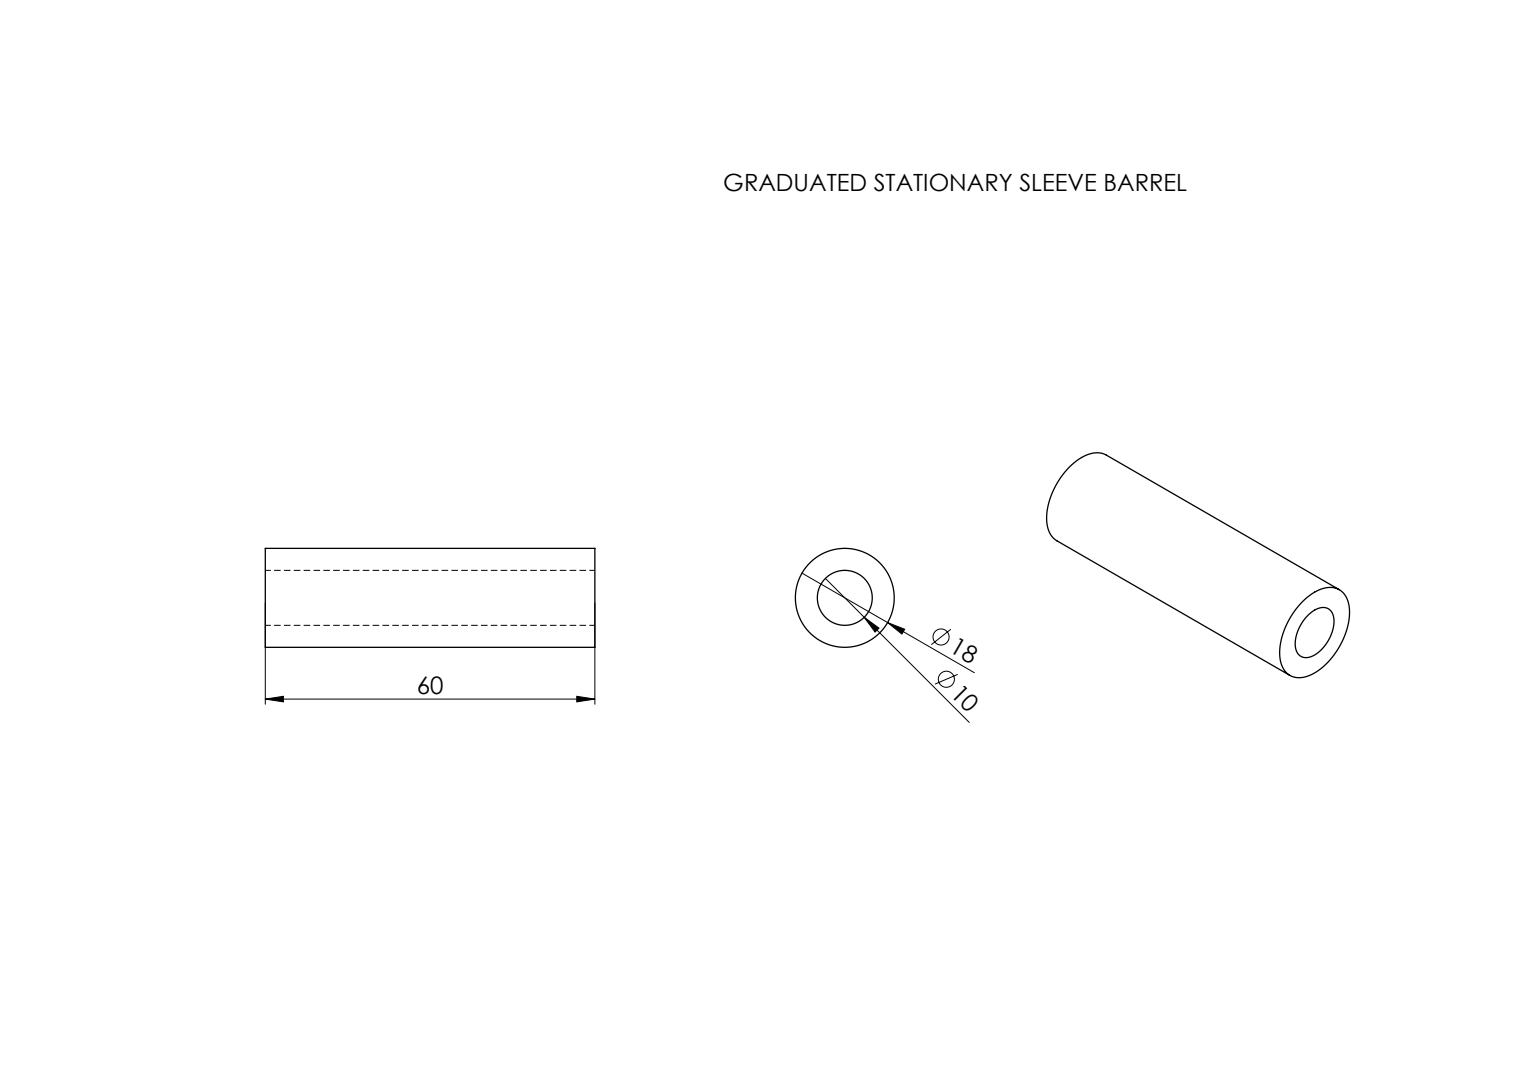
ISO-10303-21;
HEADER;
FILE_DESCRIPTION (('STEP AP214'),
    '1' );
FILE_NAME ('Graduated Stationary Sleeve Barrel.step',
    '2026-10-22T12:35:56',
    ( '' ),
    ( '' ),
    'SwSTEP 2.0',
    'SolidWorks 2026',
    '' );
FILE_SCHEMA (( 'AUTOMOTIVE_DESIGN' ));
ENDSEC;

DATA;
#3=EDGE_CURVE ( 'NONE', #403, #2721, #1745, .T. ) ;
#11=ORIENTED_EDGE ( 'NONE', *, *, #1483, .T. ) ;
#14=VECTOR ( 'NONE', #2502, 1000.000000000000000 ) ;
#17=DIRECTION ( 'NONE',  ( -0.000000000000000000, -0.000000000000000000, 1.000000000000000000 ) ) ;
#30=ORIENTED_EDGE ( 'NONE', *, *, #3, .T. ) ;
#34=DIRECTION ( 'NONE',  ( 1.000000000000000000, 2.312964634635742957E-16, 0.000000000000000000 ) ) ;
#36=CIRCLE ( 'NONE', #2432, 1.500000000000001332 ) ;
#39=DIRECTION ( 'NONE',  ( -0.000000000000000000, -0.000000000000000000, 1.000000000000000000 ) ) ;
#46=DIRECTION ( 'NONE',  ( 1.000000000000000000, 0.000000000000000000, 0.000000000000000000 ) ) ;
#48=DIRECTION ( 'NONE',  ( 0.000000000000000000, 1.000000000000000000, 0.000000000000000000 ) ) ;
#53=AXIS2_PLACEMENT_3D ( 'NONE', #2212, #1162, #2179 ) ;
#55=DIRECTION ( 'NONE',  ( -0.000000000000000000, -0.000000000000000000, 1.000000000000000000 ) ) ;
#113=DIRECTION ( 'NONE',  ( 1.000000000000000000, 0.000000000000000000, 0.000000000000000000 ) ) ;
#126=CARTESIAN_POINT ( 'NONE',  ( 38.49999999999999289, 1.474514954580286030E-14, 20.99999999999999645 ) ) ;
#133=APPLICATION_CONTEXT ( 'automotive_design' ) ;
#140=CONICAL_SURFACE ( 'NONE', #2380, 1.250000000000001110, 1.029744258676654090 ) ;
#143=CARTESIAN_POINT ( 'NONE',  ( 38.49999999999997868, 0.1985404316418196702, 16.49999999999998224 ) ) ;
#159=ORIENTED_EDGE ( 'NONE', *, *, #497, .T. ) ;
#161=AXIS2_PLACEMENT_3D ( 'NONE', #1164, #1184, #2943 ) ;
#164=FACE_OUTER_BOUND ( 'NONE', #1049, .T. ) ;
#165=ADVANCED_FACE ( 'NONE', ( #2345 ), #2393, .F. ) ;
#185=DIRECTION ( 'NONE',  ( -0.000000000000000000, -0.000000000000000000, 1.000000000000000000 ) ) ;
#191=( NAMED_UNIT ( * ) PLANE_ANGLE_UNIT ( ) SI_UNIT ( $, .RADIAN. ) );
#196=CARTESIAN_POINT ( 'NONE',  ( 35.50000000000000000, 0.1959257125632855590, 16.50000000000000000 ) ) ;
#197=ORIENTED_EDGE ( 'NONE', *, *, #540, .T. ) ;
#235=CARTESIAN_POINT ( 'NONE',  ( 38.45202114561162432, -0.3888602178275583632, 16.49210820886665374 ) ) ;
#237=CARTESIAN_POINT ( 'NONE',  ( 37.21237719682158485, -0.3527350612243344563, 12.48805154969246978 ) ) ;
#241=VERTEX_POINT ( 'NONE', #734 ) ;
#262=ORIENTED_EDGE ( 'NONE', *, *, #615, .T. ) ;
#264=EDGE_LOOP ( 'NONE', ( #371, #711 ) ) ;
#267=CARTESIAN_POINT ( 'NONE',  ( 36.63069504892280293, -0.2100771151993728880, 12.49609970571322570 ) ) ;
#268=AXIS2_PLACEMENT_3D ( 'NONE', #899, #2909, #681 ) ;
#269=CYLINDRICAL_SURFACE ( 'NONE', #1531, 1.250000000000001110 ) ;
#275=LINE ( 'NONE', #3009, #3087 ) ;
#293=ORIENTED_EDGE ( 'NONE', *, *, #2633, .T. ) ;
#294=DIRECTION ( 'NONE',  ( 1.000000000000000000, 0.000000000000000000, 0.000000000000000000 ) ) ;
#301=AXIS2_PLACEMENT_3D ( 'NONE', #323, #2823, #614 ) ;
#302=FACE_OUTER_BOUND ( 'NONE', #2160, .T. ) ;
#310=VERTEX_POINT ( 'NONE', #723 ) ;
#312=CARTESIAN_POINT ( 'NONE',  ( 37.00000000000000000, 1.474514954580286030E-14, 20.99999999999999645 ) ) ;
#318=DIRECTION ( 'NONE',  ( -1.000000000000000000, -0.000000000000000000, -0.000000000000000000 ) ) ;
#323=CARTESIAN_POINT ( 'NONE',  ( 87.00000000000000000, -7.622732162557277534E-15, 7.500000000000000000 ) ) ;
#326=VECTOR ( 'NONE', #1980, 1000.000000000000000 ) ;
#331=CARTESIAN_POINT ( 'NONE',  ( 27.00000000000000000, -7.622732162557277534E-15, 7.500000000000000000 ) ) ;
#365=CARTESIAN_POINT ( 'NONE',  ( 35.65194399346783882, -0.6651260505907211629, 16.47584948644689007 ) ) ;
#371=ORIENTED_EDGE ( 'NONE', *, *, #1189, .F. ) ;
#375=DIRECTION ( 'NONE',  ( -0.000000000000000000, -0.000000000000000000, 1.000000000000000000 ) ) ;
#379=ORIENTED_EDGE ( 'NONE', *, *, #1424, .F. ) ;
#403=VERTEX_POINT ( 'NONE', #1979 ) ;
#408=DIRECTION ( 'NONE',  ( 1.000000000000000000, 0.000000000000000000, 0.000000000000000000 ) ) ;
#416=CARTESIAN_POINT ( 'NONE',  ( 35.50000000000000000, -7.622732095468789599E-15, 16.49999999999999289 ) ) ;
#419=UNCERTAINTY_MEASURE_WITH_UNIT (LENGTH_MEASURE( 1.000000000000000082E-05 ), #2203, 'distance_accuracy_value', 'NONE');
#422=CARTESIAN_POINT ( 'NONE',  ( 38.49999999999999289, -7.622732162557277534E-15, 16.49999999999999289 ) ) ;
#423=DIRECTION ( 'NONE',  ( -3.854941057726241055E-16, 1.000000000000000000, 0.000000000000000000 ) ) ;
#429=CARTESIAN_POINT ( 'NONE',  ( 37.09819064725438409, 1.500059831078516703, 16.37410956135321882 ) ) ;
#432=ORIENTED_EDGE ( 'NONE', *, *, #882, .F. ) ;
#448=CARTESIAN_POINT ( 'NONE',  ( 38.19805860116023410, 0.9234461779904211687, 16.45357685834586903 ) ) ;
#458=( NAMED_UNIT ( * ) SI_UNIT ( $, .STERADIAN. ) SOLID_ANGLE_UNIT ( ) );
#463=DIRECTION ( 'NONE',  ( -0.000000000000000000, -0.000000000000000000, 1.000000000000000000 ) ) ;
#468=CARTESIAN_POINT ( 'NONE',  ( 38.12949724085409287, -0.9918543271721246279, 16.44544909559323287 ) ) ;
#475=ADVANCED_FACE ( 'NONE', ( #1758, #2466 ), #1952, .F. ) ;
#478=EDGE_LOOP ( 'NONE', ( #2640, #2192 ) ) ;
#481=B_SPLINE_CURVE_WITH_KNOTS ( 'NONE', 3,
 ( #609, #3129, #1643, #1588, #2584, #1338, #1883, #2554, #896, #1864 ),
 .UNSPECIFIED., .F., .F.,
 ( 4, 2, 2, 2, 4 ),
 ( 0.0002158803543021033892, 0.0005338002860526318500, 0.0008517202178031603108, 0.001169640149553688880, 0.001487560081304217232 ),
 .UNSPECIFIED. ) ;
#484=DIRECTION ( 'NONE',  ( 1.000000000000000000, 0.000000000000000000, 0.000000000000000000 ) ) ;
#489=STYLED_ITEM('',(#3271),#1054);
#497=EDGE_CURVE ( 'NONE', #2088, #3100, #2946, .T. ) ;
#507=EDGE_LOOP ( 'NONE', ( #1692, #1273, #197, #3052 ) ) ;
#512=CIRCLE ( 'NONE', #301, 8.999999999999992895 ) ;
#518=CARTESIAN_POINT ( 'NONE',  ( 38.34772064623945198, -0.6658172387807467230, 16.47579882838004295 ) ) ;
#531=VERTEX_POINT ( 'NONE', #845 ) ;
#535=VECTOR ( 'NONE', #185, 1000.000000000000000 ) ;
#540=EDGE_CURVE ( 'NONE', #2776, #241, #816, .T. ) ;
#551=AXIS2_PLACEMENT_3D ( 'NONE', #3000, #773, #2215 ) ;
#552=CARTESIAN_POINT ( 'NONE',  ( 35.80758137781342043, -0.9152444266664223615, 16.45371270176149991 ) ) ;
#567=DIRECTION ( 'NONE',  ( 0.000000000000000000, 0.000000000000000000, 1.000000000000000000 ) ) ;
#573=LINE ( 'NONE', #2313, #957 ) ;
#589=ORIENTED_EDGE ( 'NONE', *, *, #610, .T. ) ;
#603=( GEOMETRIC_REPRESENTATION_CONTEXT ( 3 ) GLOBAL_UNCERTAINTY_ASSIGNED_CONTEXT ( ( #419 ) ) GLOBAL_UNIT_ASSIGNED_CONTEXT ( ( #2203, #1706, #998 ) ) REPRESENTATION_CONTEXT ( 'NONE', 'WORKASPACE' ) );
#607=ORIENTED_EDGE ( 'NONE', *, *, #667, .F. ) ;
#609=CARTESIAN_POINT ( 'NONE',  ( 36.58213974117523293, -6.323013916343274967E-15, 12.50000000000000178 ) ) ;
#610=EDGE_CURVE ( 'NONE', #531, #1119, #1170, .T. ) ;
#611=ORIENTED_EDGE ( 'NONE', *, *, #718, .T. ) ;
#614=DIRECTION ( 'NONE',  ( 0.000000000000000000, 1.000000000000000000, 0.000000000000000000 ) ) ;
#615=EDGE_CURVE ( 'NONE', #1621, #241, #2725, .T. ) ;
#618=CIRCLE ( 'NONE', #2483, 5.000000000000000000 ) ;
#621=CARTESIAN_POINT ( 'NONE',  ( 36.58213974117523293, -6.323013916343274967E-15, 12.50000000000000178 ) ) ;
#625=CARTESIAN_POINT ( 'NONE',  ( 37.38775466693719807, 1.452318184980633031, 16.38206869443958169 ) ) ;
#630=VECTOR ( 'NONE', #2703, 1000.000000000000000 ) ;
#637=ADVANCED_FACE ( 'NONE', ( #2299 ), #812, .F. ) ;
#655=CARTESIAN_POINT ( 'NONE',  ( 37.00000000000000000, 1.474514954580286030E-14, 12.99999999999999822 ) ) ;
#661=ORIENTED_EDGE ( 'NONE', *, *, #1385, .F. ) ;
#667=EDGE_CURVE ( 'NONE', #531, #3100, #2993, .T. ) ;
#669=ORIENTED_EDGE ( 'NONE', *, *, #1688, .T. ) ;
#674=CARTESIAN_POINT ( 'NONE',  ( 87.00000000000000000, -7.622732162557277534E-15, 7.500000000000000000 ) ) ;
#676=CARTESIAN_POINT ( 'NONE',  ( 35.68903409116789049, 0.7546922429561601087, 16.47012649564898368 ) ) ;
#677=EDGE_CURVE ( 'NONE', #861, #1621, #573, .T. ) ;
#681=DIRECTION ( 'NONE',  ( 0.000000000000000000, 1.000000000000000000, 0.000000000000000000 ) ) ;
#689=CARTESIAN_POINT ( 'NONE',  ( 35.50000000000000000, -7.622732095468789599E-15, 16.49999999999999289 ) ) ;
#691=ORIENTED_EDGE ( 'NONE', *, *, #1656, .T. ) ;
#696=CARTESIAN_POINT ( 'NONE',  ( 87.00000000000000000, -7.010408762983600216E-15, 2.499999999999999556 ) ) ;
#699=CLOSED_SHELL ( 'NONE', ( #2287, #1331, #2040, #2558, #1386, #1530, #475, #2835, #165, #637, #795, #1234, #1613 ) ) ;
#704=VECTOR ( 'NONE', #1350, 1000.000000000000000 ) ;
#709=ORIENTED_EDGE ( 'NONE', *, *, #2679, .T. ) ;
#711=ORIENTED_EDGE ( 'NONE', *, *, #1812, .F. ) ;
#718=EDGE_CURVE ( 'NONE', #310, #1076, #275, .T. ) ;
#722=AXIS2_PLACEMENT_3D ( 'NONE', #2605, #1834, #113 ) ;
#723=CARTESIAN_POINT ( 'NONE',  ( 87.00000000000000000, -6.520550043324660412E-15, -1.499999999999992673 ) ) ;
#734=CARTESIAN_POINT ( 'NONE',  ( 38.25000000000000000, 1.474514954580286030E-14, 12.99999999999999822 ) ) ;
#739=AXIS2_PLACEMENT_3D ( 'NONE', #3054, #318, #567 ) ;
#742=CARTESIAN_POINT ( 'NONE',  ( 37.36887240208277916, -0.2104090322588208772, 12.49607929530250239 ) ) ;
#751=AXIS2_PLACEMENT_3D ( 'NONE', #312, #39, #294 ) ;
#757=PLANE ( 'NONE',  #2282 ) ;
#764=DIRECTION ( 'NONE',  ( 1.000000000000000000, 0.000000000000000000, 0.000000000000000000 ) ) ;
#766=DIRECTION ( 'NONE',  ( 1.000000000000000000, 0.000000000000000000, 0.000000000000000000 ) ) ;
#768=ORIENTED_EDGE ( 'NONE', *, *, #610, .F. ) ;
#773=DIRECTION ( 'NONE',  ( 1.000000000000000000, 2.312964634635742957E-16, 0.000000000000000000 ) ) ;
#775=DIRECTION ( 'NONE',  ( 1.000000000000000000, 0.000000000000000000, 0.000000000000000000 ) ) ;
#787=CARTESIAN_POINT ( 'NONE',  ( 37.41786025882473865, -0.1064896851603509553, 12.50000000000000178 ) ) ;
#795=ADVANCED_FACE ( 'NONE', ( #2578 ), #1099, .F. ) ;
#797=CIRCLE ( 'NONE', #2874, 8.999999999999992895 ) ;
#805=CARTESIAN_POINT ( 'NONE',  ( 35.75000000000000000, 1.489823039569627924E-14, 13.99999999999999822 ) ) ;
#809=COLOUR_RGB ( '',0.8941176470588234615, 0.8941176470588234615, 0.8941176470588234615 ) ;
#812=CYLINDRICAL_SURFACE ( 'NONE', #751, 1.499999999999994449 ) ;
#816=LINE ( 'NONE', #3033, #704 ) ;
#817=AXIS2_PLACEMENT_3D ( 'NONE', #2148, #3132, #1968 ) ;
#819=ORIENTED_EDGE ( 'NONE', *, *, #1576, .T. ) ;
#832=LINE ( 'NONE', #2833, #2937 ) ;
#838=LINE ( 'NONE', #2784, #2614 ) ;
#845=CARTESIAN_POINT ( 'NONE',  ( 35.50000000000000000, 1.492884656567496302E-14, 13.99999999999999822 ) ) ;
#847=ORIENTED_EDGE ( 'NONE', *, *, #1892, .F. ) ;
#850=AXIS2_PLACEMENT_3D ( 'NONE', #2539, #2547, #764 ) ;
#851=FACE_OUTER_BOUND ( 'NONE', #1488, .T. ) ;
#854=EDGE_LOOP ( 'NONE', ( #691, #589 ) ) ;
#858=EDGE_LOOP ( 'NONE', ( #30, #819 ) ) ;
#861=VERTEX_POINT ( 'NONE', #621 ) ;
#868=ORIENTED_EDGE ( 'NONE', *, *, #2571, .F. ) ;
#870=ORIENTED_EDGE ( 'NONE', *, *, #1061, .T. ) ;
#875=EDGE_LOOP ( 'NONE', ( #768, #1279, #2791, #1807 ) ) ;
#876=CARTESIAN_POINT ( 'NONE',  ( 38.49999999999999289, -7.622732162557277534E-15, 16.49999999999999289 ) ) ;
#882=EDGE_CURVE ( 'NONE', #1076, #1030, #797, .T. ) ;
#896=CARTESIAN_POINT ( 'NONE',  ( 37.41786025882475286, 0.1065494216233999342, 12.50000000000000000 ) ) ;
#898=CIRCLE ( 'NONE', #1363, 5.000000000000000000 ) ;
#899=CARTESIAN_POINT ( 'NONE',  ( 87.00000000000000000, -7.622732162557277534E-15, 7.500000000000000000 ) ) ;
#902=CARTESIAN_POINT ( 'NONE',  ( 87.00000000000000000, -7.622732162557277534E-15, 12.50000000000000000 ) ) ;
#906=AXIS2_PLACEMENT_3D ( 'NONE', #1555, #2527, #46 ) ;
#913=LINE ( 'NONE', #126, #3161 ) ;
#919=DIRECTION ( 'NONE',  ( -1.000000000000000000, -0.000000000000000000, -0.000000000000000000 ) ) ;
#932=ORIENTED_EDGE ( 'NONE', *, *, #1576, .F. ) ;
#939=AXIS2_PLACEMENT_3D ( 'NONE', #1517, #463, #766 ) ;
#942=CARTESIAN_POINT ( 'NONE',  ( 38.45998082922277916, 0.3957415549423320411, 16.49311123862705486 ) ) ;
#949=CARTESIAN_POINT ( 'NONE',  ( 38.50000000000000711, -0.09929498707317854778, 16.49999999999999645 ) ) ;
#957=VECTOR ( 'NONE', #1500, 1000.000000000000000 ) ;
#961=ORIENTED_EDGE ( 'NONE', *, *, #2571, .T. ) ;
#976=CARTESIAN_POINT ( 'NONE',  ( 38.30162487582175856, -0.7519129166725451174, 16.46890859085320002 ) ) ;
#982=( LENGTH_UNIT ( ) NAMED_UNIT ( * ) SI_UNIT ( .MILLI., .METRE. ) );
#993=FACE_OUTER_BOUND ( 'NONE', #854, .T. ) ;
#998=( NAMED_UNIT ( * ) SI_UNIT ( $, .STERADIAN. ) SOLID_ANGLE_UNIT ( ) );
#999=ORIENTED_EDGE ( 'NONE', *, *, #2679, .F. ) ;
#1011=EDGE_LOOP ( 'NONE', ( #607, #1544, #1039, #1313 ) ) ;
#1015=CARTESIAN_POINT ( 'NONE',  ( 37.41786025882474576, -7.616137346557303354E-15, 12.50000000000000000 ) ) ;
#1027=CARTESIAN_POINT ( 'NONE',  ( 35.69898883018242230, -0.7529305858385405559, 16.46882038169669471 ) ) ;
#1030=VERTEX_POINT ( 'NONE', #1461 ) ;
#1032=CARTESIAN_POINT ( 'NONE',  ( 38.50000000000000000, 1.474514954580286030E-14, 13.99999999999999822 ) ) ;
#1037=FACE_OUTER_BOUND ( 'NONE', #875, .T. ) ;
#1039=ORIENTED_EDGE ( 'NONE', *, *, #1721, .T. ) ;
#1049=EDGE_LOOP ( 'NONE', ( #11, #3163, #2385, #847, #2923, #379 ) ) ;
#1054=MANIFOLD_SOLID_BREP ( 'Boss-Extrude1', #699 ) ;
#1061=EDGE_CURVE ( 'NONE', #1916, #1595, #898, .T. ) ;
#1062=CARTESIAN_POINT ( 'NONE',  ( 36.24410157368014751, -1.310477515365985557, 16.40440676504733730 ) ) ;
#1073=CARTESIAN_POINT ( 'NONE',  ( 36.80294994545205611, -1.490236770648107001, 16.37578575999040353 ) ) ;
#1076=VERTEX_POINT ( 'NONE', #2035 ) ;
#1094=CIRCLE ( 'NONE', #161, 8.999999999999992895 ) ;
#1099=CONICAL_SURFACE ( 'NONE', #2559, 1.250000000000001110, 1.029744258676654090 ) ;
#1114=CYLINDRICAL_SURFACE ( 'NONE', #1861, 1.250000000000001110 ) ;
#1119=VERTEX_POINT ( 'NONE', #1032 ) ;
#1143=ORIENTED_EDGE ( 'NONE', *, *, #1149, .T. ) ;
#1149=EDGE_CURVE ( 'NONE', #310, #2118, #512, .T. ) ;
#1156=ORIENTED_EDGE ( 'NONE', *, *, #2976, .T. ) ;
#1162=DIRECTION ( 'NONE',  ( -1.000000000000000000, -0.000000000000000000, -0.000000000000000000 ) ) ;
#1164=CARTESIAN_POINT ( 'NONE',  ( 27.00000000000000000, -7.622732162557277534E-15, 7.500000000000000000 ) ) ;
#1170=CIRCLE ( 'NONE', #906, 1.500000000000001332 ) ;
#1177=DIRECTION ( 'NONE',  ( 0.000000000000000000, 0.000000000000000000, 1.000000000000000000 ) ) ;
#1179=CARTESIAN_POINT ( 'NONE',  ( 35.80050950286611311, 0.9216565616594220023, 16.45376772233409923 ) ) ;
#1184=DIRECTION ( 'NONE',  ( 1.000000000000000000, 2.312964634635742957E-16, 0.000000000000000000 ) ) ;
#1188=CIRCLE ( 'NONE', #2903, 5.000000000000000000 ) ;
#1189=EDGE_CURVE ( 'NONE', #2624, #2847, #1600, .T. ) ;
#1193=CARTESIAN_POINT ( 'NONE',  ( 36.60604563826974811, 1.460666791800832254, 16.38100777177577072 ) ) ;
#1217=FILL_AREA_STYLE ('',( #1245 ) ) ;
#1228=CARTESIAN_POINT ( 'NONE',  ( 37.39427925860091051, -1.460378464396907328, 16.38104908776753632 ) ) ;
#1230=CARTESIAN_POINT ( 'NONE',  ( 37.10670076043889765, -0.3922264638554286975, 12.48459209977295181 ) ) ;
#1234=ADVANCED_FACE ( 'NONE', ( #851 ), #1114, .F. ) ;
#1244=( NAMED_UNIT ( * ) PLANE_ANGLE_UNIT ( ) SI_UNIT ( $, .RADIAN. ) );
#1245=FILL_AREA_STYLE_COLOUR ( '', #809 ) ;
#1257=CARTESIAN_POINT ( 'NONE',  ( 37.00000000000000000, 1.474514954580286030E-14, 20.99999999999999645 ) ) ;
#1266=DIRECTION ( 'NONE',  ( -1.000000000000000000, -0.000000000000000000, -0.000000000000000000 ) ) ;
#1273=ORIENTED_EDGE ( 'NONE', *, *, #2997, .T. ) ;
#1279=ORIENTED_EDGE ( 'NONE', *, *, #667, .T. ) ;
#1288=CIRCLE ( 'NONE', #2072, 1.250000000000001110 ) ;
#1313=ORIENTED_EDGE ( 'NONE', *, *, #1688, .F. ) ;
#1322=CARTESIAN_POINT ( 'NONE',  ( 35.57671993710910385, -0.4836543419624433349, 16.48745487577124180 ) ) ;
#1331=ADVANCED_FACE ( 'NONE', ( #2709 ), #140, .F. ) ;
#1336=CARTESIAN_POINT ( 'NONE',  ( 36.90254329834229452, -1.500037116461185871, 16.37411340082286770 ) ) ;
#1338=CARTESIAN_POINT ( 'NONE',  ( 37.10600482971271674, 0.3921370382570182889, 12.48459913632445506 ) ) ;
#1347=DIRECTION ( 'NONE',  ( -1.000000000000000000, -0.000000000000000000, -0.000000000000000000 ) ) ;
#1350=DIRECTION ( 'NONE',  ( 0.8571673007021121116, 0.000000000000000000, 0.5150380749100544886 ) ) ;
#1363=AXIS2_PLACEMENT_3D ( 'NONE', #2734, #2249, #1546 ) ;
#1385=EDGE_CURVE ( 'NONE', #1916, #2721, #1937, .T. ) ;
#1386=ADVANCED_FACE ( 'NONE', ( #2199 ), #1426, .T. ) ;
#1390=CARTESIAN_POINT ( 'NONE',  ( 35.75000000000000000, 1.489823039569627924E-14, 20.99999999999999645 ) ) ;
#1399=CARTESIAN_POINT ( 'NONE',  ( 36.24736826332971162, 1.301195037071590122, 16.40561087244777028 ) ) ;
#1416=CARTESIAN_POINT ( 'NONE',  ( 35.53942839536622955, 0.3936020622859700002, 16.49320894598176679 ) ) ;
#1420=( GEOMETRIC_REPRESENTATION_CONTEXT ( 3 ) GLOBAL_UNCERTAINTY_ASSIGNED_CONTEXT ( ( #3107 ) ) GLOBAL_UNIT_ASSIGNED_CONTEXT ( ( #982, #1244, #2001 ) ) REPRESENTATION_CONTEXT ( 'NONE', 'WORKASPACE' ) );
#1422=PRODUCT_DEFINITION_CONTEXT ( 'detailed design', #133, 'design' ) ;
#1424=EDGE_CURVE ( 'NONE', #1595, #2776, #3151, .T. ) ;
#1425=LINE ( 'NONE', #1681, #326 ) ;
#1426=CYLINDRICAL_SURFACE ( 'NONE', #817, 8.999999999999994671 ) ;
#1429=CARTESIAN_POINT ( 'NONE',  ( 87.00000000000000000, -7.622732162557277534E-15, 16.49999999999999289 ) ) ;
#1437=ORIENTED_EDGE ( 'NONE', *, *, #2633, .F. ) ;
#1444=SHAPE_REPRESENTATION_RELATIONSHIP ( 'NONE' , 'NONE' ,  #1790, #2267 ) ;
#1461=CARTESIAN_POINT ( 'NONE',  ( 27.00000000000000000, -7.622732162557275957E-15, 16.49999999999999289 ) ) ;
#1470=CARTESIAN_POINT ( 'NONE',  ( 37.75516277711825808, -1.310683246666488833, 16.40437238582925872 ) ) ;
#1479=( LENGTH_UNIT ( ) NAMED_UNIT ( * ) SI_UNIT ( .MILLI., .METRE. ) );
#1483=EDGE_CURVE ( 'NONE', #1595, #1916, #1188, .T. ) ;
#1488=EDGE_LOOP ( 'NONE', ( #868, #2266, #709, #2653 ) ) ;
#1493=CARTESIAN_POINT ( 'NONE',  ( 36.78831377322251228, -0.3533019008417399021, 12.48801788595628892 ) ) ;
#1500=DIRECTION ( 'NONE',  ( -0.8571673007021121116, 1.049727191138618449E-16, 0.5150380749100544886 ) ) ;
#1507=CARTESIAN_POINT ( 'NONE',  ( 38.25000000000000000, 1.474514954580286030E-14, 13.99999999999999822 ) ) ;
#1510=EDGE_CURVE ( 'NONE', #241, #1621, #1288, .T. ) ;
#1517=CARTESIAN_POINT ( 'NONE',  ( 37.00000000000000000, 1.474514954580286030E-14, 13.99999999999999822 ) ) ;
#1518=DIRECTION ( 'NONE',  ( 0.000000000000000000, 1.000000000000000000, 0.000000000000000000 ) ) ;
#1523=FACE_BOUND ( 'NONE', #264, .T. ) ;
#1530=ADVANCED_FACE ( 'NONE', ( #2728, #2969 ), #2530, .T. ) ;
#1531=AXIS2_PLACEMENT_3D ( 'NONE', #1257, #1984, #2971 ) ;
#1544=ORIENTED_EDGE ( 'NONE', *, *, #1656, .F. ) ;
#1546=DIRECTION ( 'NONE',  ( 0.000000000000000000, 1.000000000000000000, 0.000000000000000000 ) ) ;
#1555=CARTESIAN_POINT ( 'NONE',  ( 37.00000000000000000, 1.474514954580286030E-14, 13.99999999999999822 ) ) ;
#1557=DIRECTION ( 'NONE',  ( -0.000000000000000000, -0.000000000000000000, 1.000000000000000000 ) ) ;
#1573=DIRECTION ( 'NONE',  ( -0.000000000000000000, -0.000000000000000000, 1.000000000000000000 ) ) ;
#1576=EDGE_CURVE ( 'NONE', #2721, #403, #618, .T. ) ;
#1577=APPLICATION_CONTEXT ( 'automotive_design' ) ;
#1587=CARTESIAN_POINT ( 'NONE',  ( 36.51683924005256188, -1.423460261948026995, 16.38679996801885252 ) ) ;
#1588=CARTESIAN_POINT ( 'NONE',  ( 36.78802102464440082, 0.3529434585571357696, 12.48803557435225287 ) ) ;
#1595=VERTEX_POINT ( 'NONE', #2790 ) ;
#1600=CIRCLE ( 'NONE', #722, 1.250000000000001110 ) ;
#1601=CARTESIAN_POINT ( 'NONE',  ( 35.49999999999999289, -0.09798730130380635395, 16.49999999999999645 ) ) ;
#1606=EDGE_CURVE ( 'NONE', #2776, #861, #3168, .T. ) ;
#1613=ADVANCED_FACE ( 'NONE', ( #1523, #993 ), #757, .F. ) ;
#1620=CARTESIAN_POINT ( 'NONE',  ( 37.91396272957889124, 1.193436492094938517, 16.42069107455876065 ) ) ;
#1621=VERTEX_POINT ( 'NONE', #3003 ) ;
#1625=DIRECTION ( 'NONE',  ( 1.000000000000000000, 0.000000000000000000, 0.000000000000000000 ) ) ;
#1643=CARTESIAN_POINT ( 'NONE',  ( 36.63137859968045262, 0.2107904407421468673, 12.49606198580778660 ) ) ;
#1647=PRODUCT ( 'Graduated Stationary Sleeve Barrel', 'Graduated Stationary Sleeve Barrel', '', ( #1938 ) ) ;
#1656=EDGE_CURVE ( 'NONE', #1119, #531, #36, .T. ) ;
#1668=DIRECTION ( 'NONE',  ( -1.000000000000000000, -0.000000000000000000, -0.000000000000000000 ) ) ;
#1681=CARTESIAN_POINT ( 'NONE',  ( 38.25000000000000000, 1.474514954580286030E-14, 20.99999999999999645 ) ) ;
#1682=CARTESIAN_POINT ( 'NONE',  ( 87.00000000000000000, -7.622732162557277534E-15, 7.500000000000000000 ) ) ;
#1688=EDGE_CURVE ( 'NONE', #3100, #2088, #1848, .T. ) ;
#1690=CARTESIAN_POINT ( 'NONE',  ( 37.48326775981566072, 1.423407605072616100, 16.38680797912481424 ) ) ;
#1692=ORIENTED_EDGE ( 'NONE', *, *, #677, .F. ) ;
#1706=( NAMED_UNIT ( * ) PLANE_ANGLE_UNIT ( ) SI_UNIT ( $, .RADIAN. ) );
#1721=EDGE_CURVE ( 'NONE', #1119, #2088, #913, .T. ) ;
#1728=CARTESIAN_POINT ( 'NONE',  ( 27.00000000000000000, -7.010408762983600216E-15, 2.499999999999999556 ) ) ;
#1732=ORIENTED_EDGE ( 'NONE', *, *, #1812, .T. ) ;
#1745=CIRCLE ( 'NONE', #1840, 5.000000000000000000 ) ;
#1758=FACE_OUTER_BOUND ( 'NONE', #1816, .T. ) ;
#1760=DIRECTION ( 'NONE',  ( -1.000000000000000000, 0.000000000000000000, -0.000000000000000000 ) ) ;
#1783=DIRECTION ( 'NONE',  ( 1.000000000000000000, 2.312964634635742957E-16, 0.000000000000000000 ) ) ;
#1788=DIRECTION ( 'NONE',  ( 0.000000000000000000, 0.000000000000000000, -1.000000000000000000 ) ) ;
#1790=SHAPE_REPRESENTATION ( 'Graduated Stationary Sleeve Barrel', ( #2878 ), #603 ) ;
#1807=ORIENTED_EDGE ( 'NONE', *, *, #1721, .F. ) ;
#1812=EDGE_CURVE ( 'NONE', #2847, #2624, #2495, .T. ) ;
#1816=EDGE_LOOP ( 'NONE', ( #3075, #432 ) ) ;
#1817=CARTESIAN_POINT ( 'NONE',  ( 36.07902659818449109, -1.200345445641969988, 16.42070378373878725 ) ) ;
#1834=DIRECTION ( 'NONE',  ( -0.000000000000000000, -0.000000000000000000, 1.000000000000000000 ) ) ;
#1837=DIRECTION ( 'NONE',  ( 1.000000000000000000, 0.000000000000000000, 0.000000000000000000 ) ) ;
#1840=AXIS2_PLACEMENT_3D ( 'NONE', #331, #1783, #1518 ) ;
#1848=B_SPLINE_CURVE_WITH_KNOTS ( 'NONE', 3,
 ( #689, #196, #1416, #676, #1179, #1942, #2920, #1399, #2365, #1193, #2652, #429, #2865, #625, #1690, #1930, #2125, #1620, #2190, #448, #3175, #942, #143, #876 ),
 .UNSPECIFIED., .F., .F.,
 ( 4, 2, 2, 2, 2, 2, 2, 2, 2, 2, 2, 4 ),
 ( 0.004697885398315436792, 0.005284974574641427766, 0.005872063750967418741, 0.006165608339130407289, 0.006459152927293394103, 0.007046242103619369465, 0.007339786691782357146, 0.007633331279945343960, 0.007926875868108331641, 0.008220420456271318455, 0.008807509632597295551, 0.009394598808923269179 ),
 .UNSPECIFIED. ) ;
#1861=AXIS2_PLACEMENT_3D ( 'NONE', #1887, #1573, #1625 ) ;
#1864=CARTESIAN_POINT ( 'NONE',  ( 37.41786025882474576, -7.616137346557303354E-15, 12.50000000000000000 ) ) ;
#1873=CYLINDRICAL_SURFACE ( 'NONE', #2446, 1.499999999999994449 ) ;
#1883=CARTESIAN_POINT ( 'NONE',  ( 37.21226234515645359, 0.3528290111407958451, 12.48804596179740756 ) ) ;
#1887=CARTESIAN_POINT ( 'NONE',  ( 37.00000000000000000, 1.474514954580286030E-14, 20.99999999999999645 ) ) ;
#1892=EDGE_CURVE ( 'NONE', #861, #403, #2205, .T. ) ;
#1897=ORIENTED_EDGE ( 'NONE', *, *, #540, .F. ) ;
#1914=ORIENTED_EDGE ( 'NONE', *, *, #718, .F. ) ;
#1916=VERTEX_POINT ( 'NONE', #2962 ) ;
#1920=UNCERTAINTY_MEASURE_WITH_UNIT (LENGTH_MEASURE( 1.000000000000000082E-05 ), #1479, 'distance_accuracy_value', 'NONE');
#1930=CARTESIAN_POINT ( 'NONE',  ( 37.66466167501430107, 1.348281052163445404, 16.39851580165995415 ) ) ;
#1932=EDGE_LOOP ( 'NONE', ( #2500, #2163, #262, #1897 ) ) ;
#1937=LINE ( 'NONE', #696, #2579 ) ;
#1938=PRODUCT_CONTEXT ( 'NONE', #1577, 'mechanical' ) ;
#1942=CARTESIAN_POINT ( 'NONE',  ( 36.00776062886353657, 1.129166992945610737, 16.42915638304272008 ) ) ;
#1952=PLANE ( 'NONE',  #551 ) ;
#1968=DIRECTION ( 'NONE',  ( 0.000000000000000000, 0.000000000000000000, 1.000000000000000000 ) ) ;
#1972=CARTESIAN_POINT ( 'NONE',  ( 27.00000000000000000, -7.622732162557277534E-15, 7.500000000000000000 ) ) ;
#1974=SURFACE_SIDE_STYLE ('',( #3190 ) ) ;
#1979=CARTESIAN_POINT ( 'NONE',  ( 27.00000000000000000, -7.622732162557277534E-15, 12.50000000000000000 ) ) ;
#1980=DIRECTION ( 'NONE',  ( -0.000000000000000000, -0.000000000000000000, 1.000000000000000000 ) ) ;
#1981=CARTESIAN_POINT ( 'NONE',  ( 36.89323119352727787, -0.3922100905875090526, 12.48459338812192776 ) ) ;
#1984=DIRECTION ( 'NONE',  ( -0.000000000000000000, -0.000000000000000000, 1.000000000000000000 ) ) ;
#1986=EDGE_LOOP ( 'NONE', ( #2461, #961, #1732, #999 ) ) ;
#1990=CIRCLE ( 'NONE', #268, 8.999999999999992895 ) ;
#2001=( NAMED_UNIT ( * ) SI_UNIT ( $, .STERADIAN. ) SOLID_ANGLE_UNIT ( ) );
#2035=CARTESIAN_POINT ( 'NONE',  ( 27.00000000000000000, -6.520550043324659623E-15, -1.499999999999992673 ) ) ;
#2036=ORIENTED_EDGE ( 'NONE', *, *, #2701, .T. ) ;
#2040=ADVANCED_FACE ( 'NONE', ( #1037 ), #1873, .F. ) ;
#2058=DIRECTION ( 'NONE',  ( 1.000000000000000000, 0.000000000000000000, 0.000000000000000000 ) ) ;
#2059=MECHANICAL_DESIGN_GEOMETRIC_PRESENTATION_REPRESENTATION('',(#2940),#3047);
#2063=CARTESIAN_POINT ( 'NONE',  ( 35.86950496355627394, -0.9908260551213471379, 16.44556929574714133 ) ) ;
#2071=CARTESIAN_POINT ( 'NONE',  ( 35.50000000000000711, 1.492884656567496302E-14, 20.99999999999999645 ) ) ;
#2072=AXIS2_PLACEMENT_3D ( 'NONE', #2758, #17, #775 ) ;
#2076=DIRECTION ( 'NONE',  ( -1.000000000000000000, -0.000000000000000000, -0.000000000000000000 ) ) ;
#2088=VERTEX_POINT ( 'NONE', #422 ) ;
#2090=CARTESIAN_POINT ( 'NONE',  ( 37.19662223785018540, -1.499925442620293259, 16.37413227714581510 ) ) ;
#2118=VERTEX_POINT ( 'NONE', #1429 ) ;
#2119=EDGE_LOOP ( 'NONE', ( #293, #1143 ) ) ;
#2125=CARTESIAN_POINT ( 'NONE',  ( 37.75078578997757717, 1.302282315510324029, 16.40545230064623183 ) ) ;
#2134=ORIENTED_EDGE ( 'NONE', *, *, #2976, .F. ) ;
#2148=CARTESIAN_POINT ( 'NONE',  ( 87.00000000000000000, -7.622732162557277534E-15, 7.500000000000000000 ) ) ;
#2160=EDGE_LOOP ( 'NONE', ( #1914, #1437, #1156, #159, #2590, #2036 ) ) ;
#2163=ORIENTED_EDGE ( 'NONE', *, *, #677, .T. ) ;
#2179=DIRECTION ( 'NONE',  ( 0.000000000000000000, 0.000000000000000000, 1.000000000000000000 ) ) ;
#2181=AXIS2_PLACEMENT_3D ( 'NONE', #2260, #2292, #2229 ) ;
#2190=CARTESIAN_POINT ( 'NONE',  ( 37.99089481476347174, 1.130332597043749665, 16.42900728359811424 ) ) ;
#2192=ORIENTED_EDGE ( 'NONE', *, *, #1061, .F. ) ;
#2199=FACE_OUTER_BOUND ( 'NONE', #3055, .T. ) ;
#2203=( LENGTH_UNIT ( ) NAMED_UNIT ( * ) SI_UNIT ( .MILLI., .METRE. ) );
#2205=LINE ( 'NONE', #2949, #630 ) ;
#2212=CARTESIAN_POINT ( 'NONE',  ( 87.00000000000000000, -7.622732162557277534E-15, 7.500000000000000000 ) ) ;
#2215=DIRECTION ( 'NONE',  ( -2.312964634635742957E-16, 1.000000000000000000, 0.000000000000000000 ) ) ;
#2217=DIRECTION ( 'NONE',  ( 1.000000000000000000, 2.312964634635742957E-16, 0.000000000000000000 ) ) ;
#2222=SURFACE_STYLE_USAGE ( .BOTH. , #1974 ) ;
#2226=ORIENTED_EDGE ( 'NONE', *, *, #1424, .T. ) ;
#2228=CARTESIAN_POINT ( 'NONE',  ( 37.41786025882474576, -7.616137346557303354E-15, 12.50000000000000000 ) ) ;
#2229=DIRECTION ( 'NONE',  ( -2.312964634635742957E-16, 1.000000000000000000, 0.000000000000000000 ) ) ;
#2245=CARTESIAN_POINT ( 'NONE',  ( 36.58213974117523293, -6.323013916343274967E-15, 12.50000000000000178 ) ) ;
#2249=DIRECTION ( 'NONE',  ( 1.000000000000000000, 2.312964634635742957E-16, 0.000000000000000000 ) ) ;
#2255=ORIENTED_EDGE ( 'NONE', *, *, #1149, .F. ) ;
#2256=EDGE_LOOP ( 'NONE', ( #661, #870, #2226, #2608, #3153, #932 ) ) ;
#2260=CARTESIAN_POINT ( 'NONE',  ( 87.00000000000000000, -7.622732162557277534E-15, 7.500000000000000000 ) ) ;
#2266=ORIENTED_EDGE ( 'NONE', *, *, #1510, .F. ) ;
#2267=ADVANCED_BREP_SHAPE_REPRESENTATION ( '', ( #1054, #2878 ), #603 ) ;
#2274=CARTESIAN_POINT ( 'NONE',  ( 38.49999999999999289, -7.622732162557277534E-15, 16.49999999999999289 ) ) ;
#2276=CARTESIAN_POINT ( 'NONE',  ( 37.00000000000000000, 1.474514954580286030E-14, 13.99999999999999822 ) ) ;
#2282=AXIS2_PLACEMENT_3D ( 'NONE', #1507, #1788, #1760 ) ;
#2287=ADVANCED_FACE ( 'NONE', ( #2747 ), #269, .F. ) ;
#2292=DIRECTION ( 'NONE',  ( 1.000000000000000000, 2.312964634635742957E-16, 0.000000000000000000 ) ) ;
#2299=FACE_OUTER_BOUND ( 'NONE', #1011, .T. ) ;
#2310=MECHANICAL_DESIGN_GEOMETRIC_PRESENTATION_REPRESENTATION('',(#489),#1420);
#2313=CARTESIAN_POINT ( 'NONE',  ( 35.75000000000000000, 1.489823039569627924E-14, 12.99999999999999822 ) ) ;
#2324=PRODUCT_DEFINITION ( 'UNKNOWN', '', #2831, #1422 ) ;
#2345=FACE_OUTER_BOUND ( 'NONE', #2256, .T. ) ;
#2365=CARTESIAN_POINT ( 'NONE',  ( 36.33339417452628339, 1.347339434735567609, 16.39865934157270289 ) ) ;
#2380=AXIS2_PLACEMENT_3D ( 'NONE', #2434, #2944, #484 ) ;
#2385=ORIENTED_EDGE ( 'NONE', *, *, #3, .F. ) ;
#2393=CYLINDRICAL_SURFACE ( 'NONE', #2512, 5.000000000000000888 ) ;
#2399=CYLINDRICAL_SURFACE ( 'NONE', #53, 5.000000000000000888 ) ;
#2432=AXIS2_PLACEMENT_3D ( 'NONE', #2276, #1557, #2541 ) ;
#2434=CARTESIAN_POINT ( 'NONE',  ( 37.00000000000000000, 1.474514954580286030E-14, 12.99999999999999822 ) ) ;
#2446=AXIS2_PLACEMENT_3D ( 'NONE', #2785, #55, #2058 ) ;
#2448=CARTESIAN_POINT ( 'NONE',  ( 38.25000000000000000, 1.474514954580286030E-14, 13.99999999999999822 ) ) ;
#2461=ORIENTED_EDGE ( 'NONE', *, *, #615, .F. ) ;
#2466=FACE_BOUND ( 'NONE', #858, .T. ) ;
#2483=AXIS2_PLACEMENT_3D ( 'NONE', #3222, #34, #48 ) ;
#2485=ORIENTED_EDGE ( 'NONE', *, *, #3208, .F. ) ;
#2495=CIRCLE ( 'NONE', #939, 1.250000000000001110 ) ;
#2500=ORIENTED_EDGE ( 'NONE', *, *, #1606, .T. ) ;
#2502=DIRECTION ( 'NONE',  ( -0.000000000000000000, -0.000000000000000000, 1.000000000000000000 ) ) ;
#2512=AXIS2_PLACEMENT_3D ( 'NONE', #674, #2649, #1177 ) ;
#2527=DIRECTION ( 'NONE',  ( -0.000000000000000000, -0.000000000000000000, 1.000000000000000000 ) ) ;
#2530=PLANE ( 'NONE',  #2181 ) ;
#2539=CARTESIAN_POINT ( 'NONE',  ( 37.00000000000000000, 1.474514954580286030E-14, 12.99999999999999822 ) ) ;
#2541=DIRECTION ( 'NONE',  ( 1.000000000000000000, 0.000000000000000000, 0.000000000000000000 ) ) ;
#2547=DIRECTION ( 'NONE',  ( -0.000000000000000000, -0.000000000000000000, 1.000000000000000000 ) ) ;
#2553=CARTESIAN_POINT ( 'NONE',  ( 35.50982285435565444, -0.1975270956567271863, 16.49834805537326687 ) ) ;
#2554=CARTESIAN_POINT ( 'NONE',  ( 37.36894289917042045, 0.2103554180567231702, 12.49608260802403237 ) ) ;
#2558=ADVANCED_FACE ( 'NONE', ( #164 ), #2399, .F. ) ;
#2559=AXIS2_PLACEMENT_3D ( 'NONE', #655, #375, #408 ) ;
#2571=EDGE_CURVE ( 'NONE', #1621, #2847, #2678, .T. ) ;
#2578=FACE_OUTER_BOUND ( 'NONE', #507, .T. ) ;
#2579=VECTOR ( 'NONE', #1668, 1000.000000000000000 ) ;
#2584=CARTESIAN_POINT ( 'NONE',  ( 36.89467617017582768, 0.3922992574225385165, 12.48458637193150089 ) ) ;
#2590=ORIENTED_EDGE ( 'NONE', *, *, #3208, .T. ) ;
#2605=CARTESIAN_POINT ( 'NONE',  ( 37.00000000000000000, 1.474514954580286030E-14, 13.99999999999999822 ) ) ;
#2608=ORIENTED_EDGE ( 'NONE', *, *, #2997, .F. ) ;
#2614=VECTOR ( 'NONE', #1347, 1000.000000000000000 ) ;
#2621=DIRECTION ( 'NONE',  ( -0.000000000000000000, -0.000000000000000000, 1.000000000000000000 ) ) ;
#2624=VERTEX_POINT ( 'NONE', #2448 ) ;
#2633=EDGE_CURVE ( 'NONE', #2118, #310, #1990, .T. ) ;
#2637=VECTOR ( 'NONE', #919, 1000.000000000000000 ) ;
#2640=ORIENTED_EDGE ( 'NONE', *, *, #1483, .F. ) ;
#2649=DIRECTION ( 'NONE',  ( -1.000000000000000000, -0.000000000000000000, -0.000000000000000000 ) ) ;
#2652=CARTESIAN_POINT ( 'NONE',  ( 36.80088933932603368, 1.499879510127410498, 16.37414004115125721 ) ) ;
#2653=ORIENTED_EDGE ( 'NONE', *, *, #1189, .T. ) ;
#2660=DIRECTION ( 'NONE',  ( 0.000000000000000000, 1.000000000000000000, 0.000000000000000000 ) ) ;
#2678=LINE ( 'NONE', #1390, #535 ) ;
#2679=EDGE_CURVE ( 'NONE', #241, #2624, #1425, .T. ) ;
#2695=CARTESIAN_POINT ( 'NONE',  ( 38.19275052663392245, -0.9148478194932491148, 16.45375607287288133 ) ) ;
#2701=EDGE_CURVE ( 'NONE', #1030, #1076, #1094, .T. ) ;
#2703=DIRECTION ( 'NONE',  ( -1.000000000000000000, -0.000000000000000000, -0.000000000000000000 ) ) ;
#2707=CARTESIAN_POINT ( 'NONE',  ( 37.92226537325434776, -1.198992358192654484, 16.42086068928975706 ) ) ;
#2709=FACE_OUTER_BOUND ( 'NONE', #1932, .T. ) ;
#2721=VERTEX_POINT ( 'NONE', #1728 ) ;
#2725=CIRCLE ( 'NONE', #850, 1.250000000000001110 ) ;
#2728=FACE_OUTER_BOUND ( 'NONE', #2119, .T. ) ;
#2734=CARTESIAN_POINT ( 'NONE',  ( 87.00000000000000000, -7.622732162557277534E-15, 7.500000000000000000 ) ) ;
#2740=ORIENTED_EDGE ( 'NONE', *, *, #882, .T. ) ;
#2746=CARTESIAN_POINT ( 'NONE',  ( 36.58213974117526845, -0.1061009270805697569, 12.50000000000000000 ) ) ;
#2747=FACE_OUTER_BOUND ( 'NONE', #1986, .T. ) ;
#2758=CARTESIAN_POINT ( 'NONE',  ( 37.00000000000000000, 1.474514954580286030E-14, 12.99999999999999822 ) ) ;
#2776=VERTEX_POINT ( 'NONE', #2228 ) ;
#2784=CARTESIAN_POINT ( 'NONE',  ( 87.00000000000000000, -7.622732162557277534E-15, 16.49999999999999289 ) ) ;
#2785=CARTESIAN_POINT ( 'NONE',  ( 37.00000000000000000, 1.474514954580286030E-14, 20.99999999999999645 ) ) ;
#2790=CARTESIAN_POINT ( 'NONE',  ( 87.00000000000000000, -7.622732162557277534E-15, 12.50000000000000000 ) ) ;
#2791=ORIENTED_EDGE ( 'NONE', *, *, #497, .F. ) ;
#2799=DIRECTION ( 'NONE',  ( 0.000000000000000000, 0.000000000000000000, 1.000000000000000000 ) ) ;
#2805=CARTESIAN_POINT ( 'NONE',  ( 35.54829862735516599, -0.3901384415568707742, 16.49205630963118807 ) ) ;
#2819=CARTESIAN_POINT ( 'NONE',  ( 35.50000000000000000, -7.622732095468789599E-15, 16.49999999999999289 ) ) ;
#2823=DIRECTION ( 'NONE',  ( 1.000000000000000000, 2.312964634635742957E-16, 0.000000000000000000 ) ) ;
#2831=PRODUCT_DEFINITION_FORMATION_WITH_SPECIFIED_SOURCE ( 'ANY', '', #1647, .NOT_KNOWN. ) ;
#2832=CARTESIAN_POINT ( 'NONE',  ( 36.61043004145795265, -1.451850406891351364, 16.38214551140935882 ) ) ;
#2833=CARTESIAN_POINT ( 'NONE',  ( 87.00000000000000000, -7.622732162557277534E-15, 16.49999999999999289 ) ) ;
#2835=ADVANCED_FACE ( 'NONE', ( #302 ), #3016, .T. ) ;
#2847=VERTEX_POINT ( 'NONE', #805 ) ;
#2865=CARTESIAN_POINT ( 'NONE',  ( 37.19571985532142122, 1.490394421081202125, 16.37575894629744866 ) ) ;
#2874=AXIS2_PLACEMENT_3D ( 'NONE', #1972, #2898, #423 ) ;
#2878=AXIS2_PLACEMENT_3D ( 'NONE', #3071, #2799, #1837 ) ;
#2898=DIRECTION ( 'NONE',  ( 1.000000000000000000, 2.312964634635742957E-16, 0.000000000000000000 ) ) ;
#2903=AXIS2_PLACEMENT_3D ( 'NONE', #1682, #2217, #2660 ) ;
#2909=DIRECTION ( 'NONE',  ( 1.000000000000000000, 2.312964634635742957E-16, 0.000000000000000000 ) ) ;
#2920=CARTESIAN_POINT ( 'NONE',  ( 36.08479696852054275, 1.192462354422088255, 16.42082098627955489 ) ) ;
#2923=ORIENTED_EDGE ( 'NONE', *, *, #1606, .F. ) ;
#2937=VECTOR ( 'NONE', #2076, 1000.000000000000000 ) ;
#2940=STYLED_ITEM ( 'NONE', ( #3207 ), #2267 ) ;
#2942=CARTESIAN_POINT ( 'NONE',  ( 38.42308964188128328, -0.4842307372812458266, 16.48742442505517047 ) ) ;
#2943=DIRECTION ( 'NONE',  ( -3.854941057726241055E-16, 1.000000000000000000, 0.000000000000000000 ) ) ;
#2944=DIRECTION ( 'NONE',  ( -0.000000000000000000, -0.000000000000000000, 1.000000000000000000 ) ) ;
#2946=B_SPLINE_CURVE_WITH_KNOTS ( 'NONE', 3,
 ( #2274, #949, #3202, #235, #2942, #518, #976, #2695, #468, #2707, #1470, #1228, #2090, #1336, #1073, #2832, #1587, #1062, #1817, #2063, #552, #1027, #365, #1322, #2805, #2553, #1601, #2819 ),
 .UNSPECIFIED., .F., .F.,
 ( 4, 2, 2, 2, 2, 2, 2, 2, 2, 2, 2, 2, 2, 4 ),
 ( 0.000000000000000000, 0.0002936178373947053669, 0.0005872356747894107339, 0.0008808535121841159924, 0.001174471349578821468, 0.001761707024368247597, 0.002348942699157674160, 0.002642560536552387117, 0.002936178373947100507, 0.003523414048736544634, 0.003817031886131267999, 0.004110649723525990930, 0.004404267560920714294, 0.004697885398315436792 ),
 .UNSPECIFIED. ) ;
#2949=CARTESIAN_POINT ( 'NONE',  ( 87.00000000000000000, -7.622732162557277534E-15, 12.50000000000000000 ) ) ;
#2962=CARTESIAN_POINT ( 'NONE',  ( 87.00000000000000000, -7.010408762983600216E-15, 2.499999999999999556 ) ) ;
#2969=FACE_BOUND ( 'NONE', #478, .T. ) ;
#2971=DIRECTION ( 'NONE',  ( 1.000000000000000000, 0.000000000000000000, 0.000000000000000000 ) ) ;
#2976=EDGE_CURVE ( 'NONE', #2118, #2088, #832, .T. ) ;
#2993=LINE ( 'NONE', #2071, #14 ) ;
#2997=EDGE_CURVE ( 'NONE', #861, #2776, #481, .T. ) ;
#3000=CARTESIAN_POINT ( 'NONE',  ( 27.00000000000000000, -7.622732162557277534E-15, 7.500000000000000000 ) ) ;
#3003=CARTESIAN_POINT ( 'NONE',  ( 35.75000000000000000, 1.489823039569627924E-14, 12.99999999999999822 ) ) ;
#3009=CARTESIAN_POINT ( 'NONE',  ( 87.00000000000000000, -6.520550043324660412E-15, -1.499999999999992673 ) ) ;
#3016=CYLINDRICAL_SURFACE ( 'NONE', #739, 8.999999999999994671 ) ;
#3033=CARTESIAN_POINT ( 'NONE',  ( 38.25000000000000000, 1.474514954580286030E-14, 12.99999999999999822 ) ) ;
#3047=( GEOMETRIC_REPRESENTATION_CONTEXT ( 3 ) GLOBAL_UNCERTAINTY_ASSIGNED_CONTEXT ( ( #1920 ) ) GLOBAL_UNIT_ASSIGNED_CONTEXT ( ( #1479, #191, #458 ) ) REPRESENTATION_CONTEXT ( 'NONE', 'WORKASPACE' ) );
#3052=ORIENTED_EDGE ( 'NONE', *, *, #1510, .T. ) ;
#3054=CARTESIAN_POINT ( 'NONE',  ( 87.00000000000000000, -7.622732162557277534E-15, 7.500000000000000000 ) ) ;
#3055=EDGE_LOOP ( 'NONE', ( #2255, #611, #2740, #2485, #669, #2134 ) ) ;
#3071=CARTESIAN_POINT ( 'NONE',  ( 0.000000000000000000, 0.000000000000000000, 0.000000000000000000 ) ) ;
#3075=ORIENTED_EDGE ( 'NONE', *, *, #2701, .F. ) ;
#3087=VECTOR ( 'NONE', #1266, 1000.000000000000000 ) ;
#3100=VERTEX_POINT ( 'NONE', #416 ) ;
#3107=UNCERTAINTY_MEASURE_WITH_UNIT (LENGTH_MEASURE( 1.000000000000000082E-05 ), #982, 'distance_accuracy_value', 'NONE');
#3129=CARTESIAN_POINT ( 'NONE',  ( 36.58213974117524714, 0.1061604454658580249, 12.49999999999999822 ) ) ;
#3132=DIRECTION ( 'NONE',  ( -1.000000000000000000, -0.000000000000000000, -0.000000000000000000 ) ) ;
#3151=LINE ( 'NONE', #902, #2637 ) ;
#3153=ORIENTED_EDGE ( 'NONE', *, *, #1892, .T. ) ;
#3161=VECTOR ( 'NONE', #2621, 1000.000000000000000 ) ;
#3163=ORIENTED_EDGE ( 'NONE', *, *, #1385, .T. ) ;
#3168=B_SPLINE_CURVE_WITH_KNOTS ( 'NONE', 3,
 ( #1015, #787, #742, #237, #1230, #1981, #1493, #267, #2746, #2245 ),
 .UNSPECIFIED., .F., .F.,
 ( 4, 2, 2, 2, 4 ),
 ( 0.001487560081304217232, 0.001805301772647892973, 0.002123043463991568930, 0.002440785155335244670, 0.002758526846678920411 ),
 .UNSPECIFIED. ) ;
#3175=CARTESIAN_POINT ( 'NONE',  ( 38.30993956269966105, 0.7564481093111570242, 16.46997477067510118 ) ) ;
#3187=SHAPE_DEFINITION_REPRESENTATION ( #3214, #1790 ) ;
#3190=SURFACE_STYLE_FILL_AREA ( #1217 ) ;
#3202=CARTESIAN_POINT ( 'NONE',  ( 38.49023808469348040, -0.1968962347057416351, 16.49835841594091690 ) ) ;
#3207=PRESENTATION_STYLE_ASSIGNMENT (( #2222 ) ) ;
#3208=EDGE_CURVE ( 'NONE', #3100, #1030, #838, .T. ) ;
#3214=PRODUCT_DEFINITION_SHAPE ( 'NONE', 'NONE',  #2324 ) ;
#3222=CARTESIAN_POINT ( 'NONE',  ( 27.00000000000000000, -7.622732162557277534E-15, 7.500000000000000000 ) ) ;
#3265=COLOUR_RGB('Off White',0.89,0.88,0.83);
#3266=FILL_AREA_STYLE_COLOUR('',#3265);
#3267=FILL_AREA_STYLE('',(#3266));
#3268=SURFACE_STYLE_FILL_AREA(#3267);
#3269=SURFACE_SIDE_STYLE('',(#3268));
#3270=SURFACE_STYLE_USAGE(.BOTH.,#3269);
#3271=PRESENTATION_STYLE_ASSIGNMENT((#3270));
ENDSEC;
END-ISO-10303-21;
